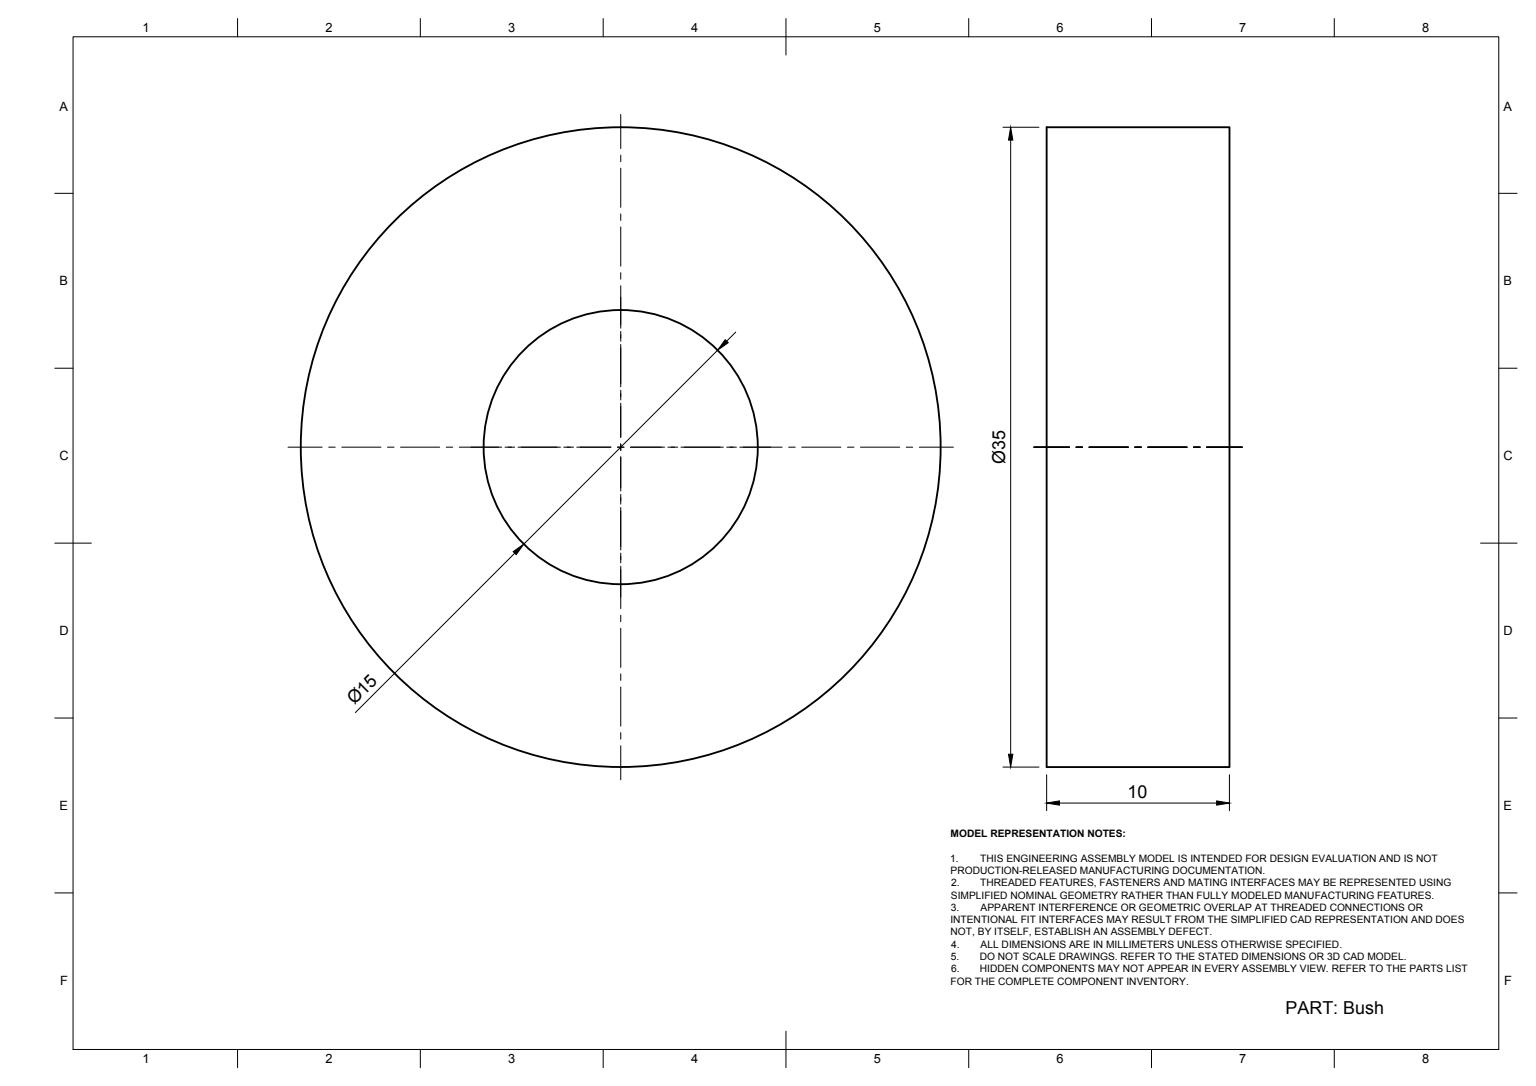
ISO-10303-21;
HEADER;
/* Generated by software containing ST-Developer
 * from STEP Tools, Inc. (www.steptools.com) 
 */

FILE_DESCRIPTION(
/* description */ ('STEP AP214'),
/* implementation_level */ '2;1');

FILE_NAME(
/* name */ 'Bush.step',
/* time_stamp */ '2026-10-05T13:15:56-07:00',
/* author */ (''),
/* organization */ (''),
/* preprocessor_version */ 'ST-DEVELOPER v20.2',
/* originating_system */ 'Autodesk Translation Framework v15.15.0.0',
/* authorisation */ '');

FILE_SCHEMA (('AUTOMOTIVE_DESIGN { 1 0 10303 214 3 1 1 }'));
ENDSEC;

DATA;
#10=MECHANICAL_DESIGN_GEOMETRIC_PRESENTATION_REPRESENTATION('',(#1356),#37881);
#1332=SHAPE_REPRESENTATION_RELATIONSHIP('SRR','None',#37965,#1344);
#1344=ADVANCED_BREP_SHAPE_REPRESENTATION('',(#1368),#37880);
#1356=STYLED_ITEM('',(#38023),#1368);
#1368=MANIFOLD_SOLID_BREP('Body1',#10830);
#1463=FACE_BOUND('',#2868,.T.);
#1464=FACE_BOUND('',#2870,.T.);
#1563=PLANE('',#11847);
#1564=PLANE('',#11848);
#2170=FACE_OUTER_BOUND('',#2865,.T.);
#2171=FACE_OUTER_BOUND('',#2866,.T.);
#2172=FACE_OUTER_BOUND('',#2867,.T.);
#2173=FACE_OUTER_BOUND('',#2869,.T.);
#2865=EDGE_LOOP('',(#10017,#10018,#10019,#10020));
#2866=EDGE_LOOP('',(#10021,#10022,#10023,#10024));
#2867=EDGE_LOOP('',(#10025));
#2868=EDGE_LOOP('',(#10026));
#2869=EDGE_LOOP('',(#10027));
#2870=EDGE_LOOP('',(#10028));
#3170=LINE('',#37803,#3471);
#3171=LINE('',#37809,#3472);
#3471=VECTOR('',#13947,7.5);
#3472=VECTOR('',#13954,17.5);
#3994=CIRCLE('',#11842,7.5);
#3995=CIRCLE('',#11843,7.5);
#3996=CIRCLE('',#11845,17.5);
#3997=CIRCLE('',#11846,17.5);
#5069=VERTEX_POINT('',#37800);
#5070=VERTEX_POINT('',#37802);
#5071=VERTEX_POINT('',#37806);
#5072=VERTEX_POINT('',#37808);
#6719=EDGE_CURVE('',#5069,#5069,#3994,.T.);
#6720=EDGE_CURVE('',#5069,#5070,#3170,.T.);
#6721=EDGE_CURVE('',#5070,#5070,#3995,.T.);
#6722=EDGE_CURVE('',#5071,#5071,#3996,.T.);
#6723=EDGE_CURVE('',#5071,#5072,#3171,.T.);
#6724=EDGE_CURVE('',#5072,#5072,#3997,.T.);
#10017=ORIENTED_EDGE('',*,*,#6719,.F.);
#10018=ORIENTED_EDGE('',*,*,#6720,.T.);
#10019=ORIENTED_EDGE('',*,*,#6721,.T.);
#10020=ORIENTED_EDGE('',*,*,#6720,.F.);
#10021=ORIENTED_EDGE('',*,*,#6722,.F.);
#10022=ORIENTED_EDGE('',*,*,#6723,.T.);
#10023=ORIENTED_EDGE('',*,*,#6724,.T.);
#10024=ORIENTED_EDGE('',*,*,#6723,.F.);
#10025=ORIENTED_EDGE('',*,*,#6722,.T.);
#10026=ORIENTED_EDGE('',*,*,#6721,.F.);
#10027=ORIENTED_EDGE('',*,*,#6724,.F.);
#10028=ORIENTED_EDGE('',*,*,#6719,.T.);
#10208=CYLINDRICAL_SURFACE('',#11841,7.5);
#10209=CYLINDRICAL_SURFACE('',#11844,17.5);
#10815=ADVANCED_FACE('',(#2170),#10208,.F.);
#10816=ADVANCED_FACE('',(#2171),#10209,.T.);
#10817=ADVANCED_FACE('',(#2172,#1463),#1563,.F.);
#10818=ADVANCED_FACE('',(#2173,#1464),#1564,.F.);
#10830=CLOSED_SHELL('',(#10815,#10816,#10817,#10818));
#11840=AXIS2_PLACEMENT_3D('',#37798,#13941,#13942);
#11841=AXIS2_PLACEMENT_3D('',#37799,#13943,#13944);
#11842=AXIS2_PLACEMENT_3D('',#37801,#13945,#13946);
#11843=AXIS2_PLACEMENT_3D('',#37804,#13948,#13949);
#11844=AXIS2_PLACEMENT_3D('',#37805,#13950,#13951);
#11845=AXIS2_PLACEMENT_3D('',#37807,#13952,#13953);
#11846=AXIS2_PLACEMENT_3D('',#37810,#13955,#13956);
#11847=AXIS2_PLACEMENT_3D('',#37811,#13957,#13958);
#11848=AXIS2_PLACEMENT_3D('',#37812,#13959,#13960);
#13941=DIRECTION('axis',(0.,0.,1.));
#13942=DIRECTION('refdir',(1.,0.,0.));
#13943=DIRECTION('center_axis',(1.49883571991992E-29,3.54987407349455E-30,
1.));
#13944=DIRECTION('ref_axis',(1.,-1.26016059376688E-58,-1.49883571991992E-29));
#13945=DIRECTION('center_axis',(1.49883571991992E-29,3.54987407349455E-30,
1.));
#13946=DIRECTION('ref_axis',(1.,-5.32067806257128E-59,-1.49883571991992E-29));
#13947=DIRECTION('',(1.49883571991992E-29,3.54987407349455E-30,1.));
#13948=DIRECTION('center_axis',(1.49883571991992E-29,3.54987407349455E-30,
1.));
#13949=DIRECTION('ref_axis',(1.,-1.26016059376688E-58,-1.49883571991992E-29));
#13950=DIRECTION('center_axis',(1.49883571991992E-29,3.54987407349455E-30,
1.));
#13951=DIRECTION('ref_axis',(1.,-1.26016059376688E-58,-1.49883571991992E-29));
#13952=DIRECTION('center_axis',(1.49883571991992E-29,3.54987407349455E-30,
1.));
#13953=DIRECTION('ref_axis',(1.,-1.26016059376688E-58,-1.49883571991992E-29));
#13954=DIRECTION('',(-1.49883571991992E-29,-3.54987407349455E-30,-1.));
#13955=DIRECTION('center_axis',(1.49883571991992E-29,3.54987407349455E-30,
1.));
#13956=DIRECTION('ref_axis',(1.,-5.32067806257128E-59,-1.49883571991992E-29));
#13957=DIRECTION('center_axis',(2.05103835357463E-29,-3.54987407349455E-30,
-1.));
#13958=DIRECTION('ref_axis',(-1.,0.,-2.05103835357463E-29));
#13959=DIRECTION('center_axis',(-2.05103835357463E-29,3.54987407349455E-30,
1.));
#13960=DIRECTION('ref_axis',(1.,0.,2.05103835357463E-29));
#37798=CARTESIAN_POINT('',(0.,0.,0.));
#37799=CARTESIAN_POINT('Origin',(0.,0.,0.));
#37800=CARTESIAN_POINT('',(-7.5,-9.1848509936055E-16,-10.));
#37801=CARTESIAN_POINT('Origin',(0.,-1.38777878078145E-14,-10.));
#37802=CARTESIAN_POINT('',(-7.5,-9.18485099360515E-16,1.12412678993994E-28));
#37803=CARTESIAN_POINT('',(-7.5,-9.18485099360515E-16,1.12412678993994E-28));
#37804=CARTESIAN_POINT('Origin',(0.,0.,0.));
#37805=CARTESIAN_POINT('Origin',(0.,0.,0.));
#37806=CARTESIAN_POINT('',(-17.5,-2.14313189850787E-15,2.62296250985986E-28));
#37807=CARTESIAN_POINT('Origin',(0.,0.,0.));
#37808=CARTESIAN_POINT('',(-17.5,-2.1431318985079E-15,-10.));
#37809=CARTESIAN_POINT('',(-17.5,-2.14313189850787E-15,2.62296250985986E-28));
#37810=CARTESIAN_POINT('Origin',(0.,-1.38777878078145E-14,-10.));
#37811=CARTESIAN_POINT('Origin',(0.,7.5,0.));
#37812=CARTESIAN_POINT('Origin',(0.,7.5,-10.));
#37866=UNCERTAINTY_MEASURE_WITH_UNIT(LENGTH_MEASURE(0.01),#37882,
'DISTANCE_ACCURACY_VALUE',
'Maximum model space distance between geometric entities at asserted c
onnectivities');
#37867=UNCERTAINTY_MEASURE_WITH_UNIT(LENGTH_MEASURE(0.01),#37882,
'DISTANCE_ACCURACY_VALUE',
'Maximum model space distance between geometric entities at asserted c
onnectivities');
#37880=(
GEOMETRIC_REPRESENTATION_CONTEXT(3)
GLOBAL_UNCERTAINTY_ASSIGNED_CONTEXT((#37866))
GLOBAL_UNIT_ASSIGNED_CONTEXT((#37882,#37884,#37885))
REPRESENTATION_CONTEXT('','3D')
);
#37881=(
GEOMETRIC_REPRESENTATION_CONTEXT(3)
GLOBAL_UNCERTAINTY_ASSIGNED_CONTEXT((#37867))
GLOBAL_UNIT_ASSIGNED_CONTEXT((#37882,#37884,#37885))
REPRESENTATION_CONTEXT('','3D')
);
#37882=(
LENGTH_UNIT()
NAMED_UNIT(*)
SI_UNIT(.MILLI.,.METRE.)
);
#37884=(
NAMED_UNIT(*)
PLANE_ANGLE_UNIT()
SI_UNIT($,.RADIAN.)
);
#37885=(
NAMED_UNIT(*)
SI_UNIT($,.STERADIAN.)
SOLID_ANGLE_UNIT()
);
#37898=SHAPE_DEFINITION_REPRESENTATION(#37911,#37965);
#37911=PRODUCT_DEFINITION_SHAPE('',$,#37979);
#37965=SHAPE_REPRESENTATION('',(#11840),#37880);
#37966=PRODUCT_DEFINITION_CONTEXT('part definition',#38007,'design');
#37979=PRODUCT_DEFINITION('PS12','Bush',#37992,#37966);
#37992=PRODUCT_DEFINITION_FORMATION('',$,#38021);
#38007=APPLICATION_CONTEXT(
'Core Data for Automotive Mechanical Design Process');
#38008=PRODUCT_CONTEXT('part definition',#38007,'mechanical');
#38021=PRODUCT('PS12','Bush',$,(#38008));
#38023=PRESENTATION_STYLE_ASSIGNMENT((#38025));
#38025=SURFACE_STYLE_USAGE(.BOTH.,#38027);
#38027=SURFACE_SIDE_STYLE('',(#38029));
#38029=SURFACE_STYLE_FILL_AREA(#38031);
#38031=FILL_AREA_STYLE('Opaque(202,209,238)',(#38033));
#38033=FILL_AREA_STYLE_COLOUR('Opaque(202,209,238)',#38035);
#38035=COLOUR_RGB('Opaque(202,209,238)', 0.66274510, 0.83137255, 0.94901961);
ENDSEC;
END-ISO-10303-21;
